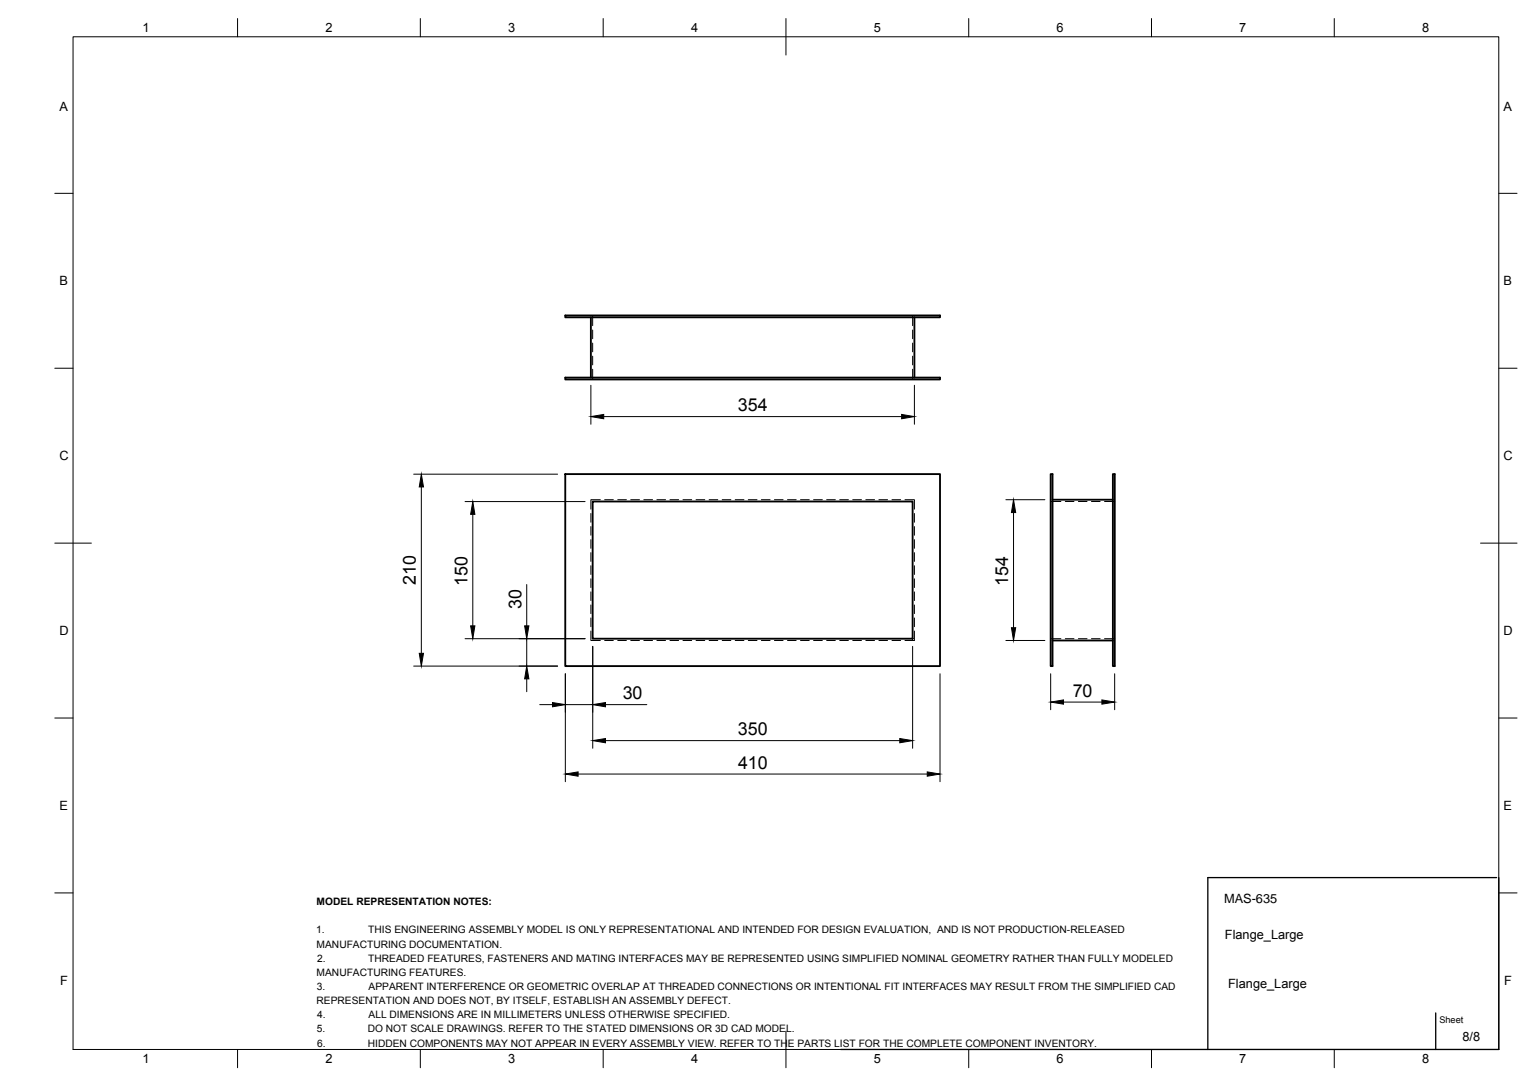
ISO-10303-21;
HEADER;
FILE_DESCRIPTION((''),'2;1');
FILE_NAME('Flange_Large.step','2026-10-09T12:34:24-07:00',(''),(''),'','','');
FILE_SCHEMA (('AUTOMOTIVE_DESIGN { 1 0 10303 214 3 1 1 }'));
ENDSEC;
DATA;
#10=MECHANICAL_DESIGN_GEOMETRIC_PRESENTATION_REPRESENTATION('',(#63),#3759);
#51=SHAPE_REPRESENTATION_RELATIONSHIP('SRR','None',#3792,#57) ;
#57=ADVANCED_BREP_SHAPE_REPRESENTATION('',(#69),#3757) ;
#63=STYLED_ITEM('',(#3827),#69) ;
#69=MANIFOLD_SOLID_BREP('Body1',#2267) ;
#133=FACE_BOUND('',#360,.T.) ;
#134=FACE_BOUND('',#362,.T.) ;
#135=FACE_BOUND('',#372,.T.) ;
#136=FACE_BOUND('',#374,.T.) ;
#221=FACE_OUTER_BOUND('',#355,.T.) ;
#222=FACE_OUTER_BOUND('',#356,.T.) ;
#223=FACE_OUTER_BOUND('',#357,.T.) ;
#224=FACE_OUTER_BOUND('',#358,.T.) ;
#225=FACE_OUTER_BOUND('',#359,.T.) ;
#226=FACE_OUTER_BOUND('',#361,.T.) ;
#227=FACE_OUTER_BOUND('',#363,.T.) ;
#228=FACE_OUTER_BOUND('',#364,.T.) ;
#229=FACE_OUTER_BOUND('',#365,.T.) ;
#230=FACE_OUTER_BOUND('',#366,.T.) ;
#231=FACE_OUTER_BOUND('',#367,.T.) ;
#232=FACE_OUTER_BOUND('',#368,.T.) ;
#233=FACE_OUTER_BOUND('',#369,.T.) ;
#234=FACE_OUTER_BOUND('',#370,.T.) ;
#235=FACE_OUTER_BOUND('',#371,.T.) ;
#236=FACE_OUTER_BOUND('',#373,.T.) ;
#237=FACE_OUTER_BOUND('',#375,.T.) ;
#238=FACE_OUTER_BOUND('',#376,.T.) ;
#239=FACE_OUTER_BOUND('',#377,.T.) ;
#240=FACE_OUTER_BOUND('',#378,.T.) ;
#355=EDGE_LOOP('',(#1847,#1848,#1849,#1850)) ;
#356=EDGE_LOOP('',(#1851,#1852,#1853,#1854)) ;
#357=EDGE_LOOP('',(#1855,#1856,#1857,#1858)) ;
#358=EDGE_LOOP('',(#1859,#1860,#1861,#1862)) ;
#359=EDGE_LOOP('',(#1863,#1864,#1865,#1866)) ;
#360=EDGE_LOOP('',(#1867,#1868,#1869,#1870)) ;
#361=EDGE_LOOP('',(#1871,#1872,#1873,#1874)) ;
#362=EDGE_LOOP('',(#1875,#1876,#1877,#1878)) ;
#363=EDGE_LOOP('',(#1879,#1880,#1881,#1882)) ;
#364=EDGE_LOOP('',(#1883,#1884,#1885,#1886)) ;
#365=EDGE_LOOP('',(#1887,#1888,#1889,#1890)) ;
#366=EDGE_LOOP('',(#1891,#1892,#1893,#1894)) ;
#367=EDGE_LOOP('',(#1895,#1896,#1897,#1898)) ;
#368=EDGE_LOOP('',(#1899,#1900,#1901,#1902)) ;
#369=EDGE_LOOP('',(#1903,#1904,#1905,#1906)) ;
#370=EDGE_LOOP('',(#1907,#1908,#1909,#1910)) ;
#371=EDGE_LOOP('',(#1911,#1912,#1913,#1914)) ;
#372=EDGE_LOOP('',(#1915,#1916,#1917,#1918)) ;
#373=EDGE_LOOP('',(#1919,#1920,#1921,#1922)) ;
#374=EDGE_LOOP('',(#1923,#1924,#1925,#1926)) ;
#375=EDGE_LOOP('',(#1927,#1928,#1929,#1930)) ;
#376=EDGE_LOOP('',(#1931,#1932,#1933,#1934)) ;
#377=EDGE_LOOP('',(#1935,#1936,#1937,#1938)) ;
#378=EDGE_LOOP('',(#1939,#1940,#1941,#1942)) ;
#575=LINE('',#3537,#843) ;
#576=LINE('',#3539,#844) ;
#577=LINE('',#3541,#845) ;
#578=LINE('',#3542,#846) ;
#579=LINE('',#3545,#847) ;
#580=LINE('',#3547,#848) ;
#581=LINE('',#3548,#849) ;
#582=LINE('',#3551,#850) ;
#583=LINE('',#3553,#851) ;
#584=LINE('',#3554,#852) ;
#585=LINE('',#3556,#853) ;
#586=LINE('',#3557,#854) ;
#587=LINE('',#3561,#855) ;
#588=LINE('',#3563,#856) ;
#589=LINE('',#3565,#857) ;
#590=LINE('',#3566,#858) ;
#591=LINE('',#3570,#859) ;
#592=LINE('',#3572,#860) ;
#593=LINE('',#3574,#861) ;
#594=LINE('',#3575,#862) ;
#595=LINE('',#3578,#863) ;
#596=LINE('',#3580,#864) ;
#597=LINE('',#3582,#865) ;
#598=LINE('',#3583,#866) ;
#599=LINE('',#3585,#867) ;
#600=LINE('',#3586,#868) ;
#601=LINE('',#3588,#869) ;
#602=LINE('',#3590,#870) ;
#603=LINE('',#3594,#871) ;
#604=LINE('',#3596,#872) ;
#605=LINE('',#3597,#873) ;
#606=LINE('',#3600,#874) ;
#607=LINE('',#3601,#875) ;
#608=LINE('',#3604,#876) ;
#609=LINE('',#3605,#877) ;
#610=LINE('',#3607,#878) ;
#611=LINE('',#3611,#879) ;
#612=LINE('',#3613,#880) ;
#613=LINE('',#3615,#881) ;
#614=LINE('',#3616,#882) ;
#615=LINE('',#3620,#883) ;
#616=LINE('',#3622,#884) ;
#617=LINE('',#3624,#885) ;
#618=LINE('',#3625,#886) ;
#619=LINE('',#3627,#887) ;
#620=LINE('',#3628,#888) ;
#621=LINE('',#3630,#889) ;
#622=LINE('',#3632,#890) ;
#843=VECTOR('',#2914,100.) ;
#844=VECTOR('',#2915,100.) ;
#845=VECTOR('',#2916,100.) ;
#846=VECTOR('',#2917,100.) ;
#847=VECTOR('',#2920,100.) ;
#848=VECTOR('',#2921,100.) ;
#849=VECTOR('',#2922,100.) ;
#850=VECTOR('',#2925,100.) ;
#851=VECTOR('',#2926,100.) ;
#852=VECTOR('',#2927,100.) ;
#853=VECTOR('',#2930,100.) ;
#854=VECTOR('',#2931,100.) ;
#855=VECTOR('',#2934,100.) ;
#856=VECTOR('',#2935,100.) ;
#857=VECTOR('',#2936,100.) ;
#858=VECTOR('',#2937,100.) ;
#859=VECTOR('',#2940,100.) ;
#860=VECTOR('',#2941,100.) ;
#861=VECTOR('',#2942,100.) ;
#862=VECTOR('',#2943,100.) ;
#863=VECTOR('',#2944,100.) ;
#864=VECTOR('',#2945,100.) ;
#865=VECTOR('',#2946,100.) ;
#866=VECTOR('',#2947,100.) ;
#867=VECTOR('',#2950,100.) ;
#868=VECTOR('',#2951,100.) ;
#869=VECTOR('',#2954,100.) ;
#870=VECTOR('',#2957,100.) ;
#871=VECTOR('',#2962,100.) ;
#872=VECTOR('',#2963,100.) ;
#873=VECTOR('',#2964,100.) ;
#874=VECTOR('',#2967,100.) ;
#875=VECTOR('',#2968,100.) ;
#876=VECTOR('',#2971,100.) ;
#877=VECTOR('',#2972,100.) ;
#878=VECTOR('',#2975,100.) ;
#879=VECTOR('',#2978,100.) ;
#880=VECTOR('',#2979,100.) ;
#881=VECTOR('',#2980,100.) ;
#882=VECTOR('',#2981,100.) ;
#883=VECTOR('',#2984,100.) ;
#884=VECTOR('',#2985,100.) ;
#885=VECTOR('',#2986,100.) ;
#886=VECTOR('',#2987,100.) ;
#887=VECTOR('',#2990,100.) ;
#888=VECTOR('',#2991,100.) ;
#889=VECTOR('',#2994,100.) ;
#890=VECTOR('',#2997,100.) ;
#1075=VERTEX_POINT('',#3535) ;
#1076=VERTEX_POINT('',#3536) ;
#1077=VERTEX_POINT('',#3538) ;
#1078=VERTEX_POINT('',#3540) ;
#1079=VERTEX_POINT('',#3544) ;
#1080=VERTEX_POINT('',#3546) ;
#1081=VERTEX_POINT('',#3550) ;
#1082=VERTEX_POINT('',#3552) ;
#1083=VERTEX_POINT('',#3559) ;
#1084=VERTEX_POINT('',#3560) ;
#1085=VERTEX_POINT('',#3562) ;
#1086=VERTEX_POINT('',#3564) ;
#1087=VERTEX_POINT('',#3568) ;
#1088=VERTEX_POINT('',#3569) ;
#1089=VERTEX_POINT('',#3571) ;
#1090=VERTEX_POINT('',#3573) ;
#1091=VERTEX_POINT('',#3576) ;
#1092=VERTEX_POINT('',#3577) ;
#1093=VERTEX_POINT('',#3579) ;
#1094=VERTEX_POINT('',#3581) ;
#1095=VERTEX_POINT('',#3593) ;
#1096=VERTEX_POINT('',#3595) ;
#1097=VERTEX_POINT('',#3599) ;
#1098=VERTEX_POINT('',#3603) ;
#1099=VERTEX_POINT('',#3609) ;
#1100=VERTEX_POINT('',#3610) ;
#1101=VERTEX_POINT('',#3612) ;
#1102=VERTEX_POINT('',#3614) ;
#1103=VERTEX_POINT('',#3618) ;
#1104=VERTEX_POINT('',#3619) ;
#1105=VERTEX_POINT('',#3621) ;
#1106=VERTEX_POINT('',#3623) ;
#1343=EDGE_CURVE('',#1075,#1076,#575,.T.) ;
#1344=EDGE_CURVE('',#1075,#1077,#576,.T.) ;
#1345=EDGE_CURVE('',#1078,#1077,#577,.T.) ;
#1346=EDGE_CURVE('',#1076,#1078,#578,.T.) ;
#1347=EDGE_CURVE('',#1076,#1079,#579,.T.) ;
#1348=EDGE_CURVE('',#1080,#1078,#580,.T.) ;
#1349=EDGE_CURVE('',#1079,#1080,#581,.T.) ;
#1350=EDGE_CURVE('',#1079,#1081,#582,.T.) ;
#1351=EDGE_CURVE('',#1082,#1080,#583,.T.) ;
#1352=EDGE_CURVE('',#1081,#1082,#584,.T.) ;
#1353=EDGE_CURVE('',#1081,#1075,#585,.T.) ;
#1354=EDGE_CURVE('',#1077,#1082,#586,.T.) ;
#1355=EDGE_CURVE('',#1083,#1084,#587,.T.) ;
#1356=EDGE_CURVE('',#1084,#1085,#588,.T.) ;
#1357=EDGE_CURVE('',#1085,#1086,#589,.T.) ;
#1358=EDGE_CURVE('',#1086,#1083,#590,.T.) ;
#1359=EDGE_CURVE('',#1087,#1088,#591,.T.) ;
#1360=EDGE_CURVE('',#1089,#1087,#592,.T.) ;
#1361=EDGE_CURVE('',#1090,#1089,#593,.T.) ;
#1362=EDGE_CURVE('',#1088,#1090,#594,.T.) ;
#1363=EDGE_CURVE('',#1091,#1092,#595,.T.) ;
#1364=EDGE_CURVE('',#1092,#1093,#596,.T.) ;
#1365=EDGE_CURVE('',#1093,#1094,#597,.T.) ;
#1366=EDGE_CURVE('',#1094,#1091,#598,.T.) ;
#1367=EDGE_CURVE('',#1084,#1088,#599,.T.) ;
#1368=EDGE_CURVE('',#1083,#1087,#600,.T.) ;
#1369=EDGE_CURVE('',#1085,#1090,#601,.T.) ;
#1370=EDGE_CURVE('',#1086,#1089,#602,.T.) ;
#1371=EDGE_CURVE('',#1095,#1092,#603,.T.) ;
#1372=EDGE_CURVE('',#1096,#1091,#604,.T.) ;
#1373=EDGE_CURVE('',#1096,#1095,#605,.T.) ;
#1374=EDGE_CURVE('',#1097,#1093,#606,.T.) ;
#1375=EDGE_CURVE('',#1095,#1097,#607,.T.) ;
#1376=EDGE_CURVE('',#1098,#1094,#608,.T.) ;
#1377=EDGE_CURVE('',#1097,#1098,#609,.T.) ;
#1378=EDGE_CURVE('',#1098,#1096,#610,.T.) ;
#1379=EDGE_CURVE('',#1099,#1100,#611,.T.) ;
#1380=EDGE_CURVE('',#1100,#1101,#612,.T.) ;
#1381=EDGE_CURVE('',#1101,#1102,#613,.T.) ;
#1382=EDGE_CURVE('',#1102,#1099,#614,.T.) ;
#1383=EDGE_CURVE('',#1103,#1104,#615,.T.) ;
#1384=EDGE_CURVE('',#1105,#1103,#616,.T.) ;
#1385=EDGE_CURVE('',#1106,#1105,#617,.T.) ;
#1386=EDGE_CURVE('',#1104,#1106,#618,.T.) ;
#1387=EDGE_CURVE('',#1103,#1099,#619,.T.) ;
#1388=EDGE_CURVE('',#1104,#1100,#620,.T.) ;
#1389=EDGE_CURVE('',#1105,#1102,#621,.T.) ;
#1390=EDGE_CURVE('',#1106,#1101,#622,.T.) ;
#1847=ORIENTED_EDGE('',*,*,#1343,.F.) ;
#1848=ORIENTED_EDGE('',*,*,#1344,.T.) ;
#1849=ORIENTED_EDGE('',*,*,#1345,.F.) ;
#1850=ORIENTED_EDGE('',*,*,#1346,.F.) ;
#1851=ORIENTED_EDGE('',*,*,#1347,.F.) ;
#1852=ORIENTED_EDGE('',*,*,#1346,.T.) ;
#1853=ORIENTED_EDGE('',*,*,#1348,.F.) ;
#1854=ORIENTED_EDGE('',*,*,#1349,.F.) ;
#1855=ORIENTED_EDGE('',*,*,#1350,.F.) ;
#1856=ORIENTED_EDGE('',*,*,#1349,.T.) ;
#1857=ORIENTED_EDGE('',*,*,#1351,.F.) ;
#1858=ORIENTED_EDGE('',*,*,#1352,.F.) ;
#1859=ORIENTED_EDGE('',*,*,#1353,.F.) ;
#1860=ORIENTED_EDGE('',*,*,#1352,.T.) ;
#1861=ORIENTED_EDGE('',*,*,#1354,.F.) ;
#1862=ORIENTED_EDGE('',*,*,#1344,.F.) ;
#1863=ORIENTED_EDGE('',*,*,#1355,.T.) ;
#1864=ORIENTED_EDGE('',*,*,#1356,.T.) ;
#1865=ORIENTED_EDGE('',*,*,#1357,.T.) ;
#1866=ORIENTED_EDGE('',*,*,#1358,.T.) ;
#1867=ORIENTED_EDGE('',*,*,#1348,.T.) ;
#1868=ORIENTED_EDGE('',*,*,#1345,.T.) ;
#1869=ORIENTED_EDGE('',*,*,#1354,.T.) ;
#1870=ORIENTED_EDGE('',*,*,#1351,.T.) ;
#1871=ORIENTED_EDGE('',*,*,#1359,.F.) ;
#1872=ORIENTED_EDGE('',*,*,#1360,.F.) ;
#1873=ORIENTED_EDGE('',*,*,#1361,.F.) ;
#1874=ORIENTED_EDGE('',*,*,#1362,.F.) ;
#1875=ORIENTED_EDGE('',*,*,#1363,.T.) ;
#1876=ORIENTED_EDGE('',*,*,#1364,.T.) ;
#1877=ORIENTED_EDGE('',*,*,#1365,.T.) ;
#1878=ORIENTED_EDGE('',*,*,#1366,.T.) ;
#1879=ORIENTED_EDGE('',*,*,#1359,.T.) ;
#1880=ORIENTED_EDGE('',*,*,#1367,.F.) ;
#1881=ORIENTED_EDGE('',*,*,#1355,.F.) ;
#1882=ORIENTED_EDGE('',*,*,#1368,.T.) ;
#1883=ORIENTED_EDGE('',*,*,#1362,.T.) ;
#1884=ORIENTED_EDGE('',*,*,#1369,.F.) ;
#1885=ORIENTED_EDGE('',*,*,#1356,.F.) ;
#1886=ORIENTED_EDGE('',*,*,#1367,.T.) ;
#1887=ORIENTED_EDGE('',*,*,#1361,.T.) ;
#1888=ORIENTED_EDGE('',*,*,#1370,.F.) ;
#1889=ORIENTED_EDGE('',*,*,#1357,.F.) ;
#1890=ORIENTED_EDGE('',*,*,#1369,.T.) ;
#1891=ORIENTED_EDGE('',*,*,#1360,.T.) ;
#1892=ORIENTED_EDGE('',*,*,#1368,.F.) ;
#1893=ORIENTED_EDGE('',*,*,#1358,.F.) ;
#1894=ORIENTED_EDGE('',*,*,#1370,.T.) ;
#1895=ORIENTED_EDGE('',*,*,#1371,.T.) ;
#1896=ORIENTED_EDGE('',*,*,#1363,.F.) ;
#1897=ORIENTED_EDGE('',*,*,#1372,.F.) ;
#1898=ORIENTED_EDGE('',*,*,#1373,.T.) ;
#1899=ORIENTED_EDGE('',*,*,#1374,.T.) ;
#1900=ORIENTED_EDGE('',*,*,#1364,.F.) ;
#1901=ORIENTED_EDGE('',*,*,#1371,.F.) ;
#1902=ORIENTED_EDGE('',*,*,#1375,.T.) ;
#1903=ORIENTED_EDGE('',*,*,#1376,.T.) ;
#1904=ORIENTED_EDGE('',*,*,#1365,.F.) ;
#1905=ORIENTED_EDGE('',*,*,#1374,.F.) ;
#1906=ORIENTED_EDGE('',*,*,#1377,.T.) ;
#1907=ORIENTED_EDGE('',*,*,#1372,.T.) ;
#1908=ORIENTED_EDGE('',*,*,#1366,.F.) ;
#1909=ORIENTED_EDGE('',*,*,#1376,.F.) ;
#1910=ORIENTED_EDGE('',*,*,#1378,.T.) ;
#1911=ORIENTED_EDGE('',*,*,#1379,.T.) ;
#1912=ORIENTED_EDGE('',*,*,#1380,.T.) ;
#1913=ORIENTED_EDGE('',*,*,#1381,.T.) ;
#1914=ORIENTED_EDGE('',*,*,#1382,.T.) ;
#1915=ORIENTED_EDGE('',*,*,#1375,.F.) ;
#1916=ORIENTED_EDGE('',*,*,#1373,.F.) ;
#1917=ORIENTED_EDGE('',*,*,#1378,.F.) ;
#1918=ORIENTED_EDGE('',*,*,#1377,.F.) ;
#1919=ORIENTED_EDGE('',*,*,#1383,.F.) ;
#1920=ORIENTED_EDGE('',*,*,#1384,.F.) ;
#1921=ORIENTED_EDGE('',*,*,#1385,.F.) ;
#1922=ORIENTED_EDGE('',*,*,#1386,.F.) ;
#1923=ORIENTED_EDGE('',*,*,#1353,.T.) ;
#1924=ORIENTED_EDGE('',*,*,#1343,.T.) ;
#1925=ORIENTED_EDGE('',*,*,#1347,.T.) ;
#1926=ORIENTED_EDGE('',*,*,#1350,.T.) ;
#1927=ORIENTED_EDGE('',*,*,#1379,.F.) ;
#1928=ORIENTED_EDGE('',*,*,#1387,.F.) ;
#1929=ORIENTED_EDGE('',*,*,#1383,.T.) ;
#1930=ORIENTED_EDGE('',*,*,#1388,.T.) ;
#1931=ORIENTED_EDGE('',*,*,#1382,.F.) ;
#1932=ORIENTED_EDGE('',*,*,#1389,.F.) ;
#1933=ORIENTED_EDGE('',*,*,#1384,.T.) ;
#1934=ORIENTED_EDGE('',*,*,#1387,.T.) ;
#1935=ORIENTED_EDGE('',*,*,#1381,.F.) ;
#1936=ORIENTED_EDGE('',*,*,#1390,.F.) ;
#1937=ORIENTED_EDGE('',*,*,#1385,.T.) ;
#1938=ORIENTED_EDGE('',*,*,#1389,.T.) ;
#1939=ORIENTED_EDGE('',*,*,#1380,.F.) ;
#1940=ORIENTED_EDGE('',*,*,#1388,.F.) ;
#1941=ORIENTED_EDGE('',*,*,#1386,.T.) ;
#1942=ORIENTED_EDGE('',*,*,#1390,.T.) ;
#2103=PLANE('',#2454) ;
#2104=PLANE('',#2455) ;
#2105=PLANE('',#2456) ;
#2106=PLANE('',#2457) ;
#2107=PLANE('',#2458) ;
#2108=PLANE('',#2459) ;
#2109=PLANE('',#2460) ;
#2110=PLANE('',#2461) ;
#2111=PLANE('',#2462) ;
#2112=PLANE('',#2463) ;
#2113=PLANE('',#2464) ;
#2114=PLANE('',#2465) ;
#2115=PLANE('',#2466) ;
#2116=PLANE('',#2467) ;
#2117=PLANE('',#2468) ;
#2118=PLANE('',#2469) ;
#2119=PLANE('',#2470) ;
#2120=PLANE('',#2471) ;
#2121=PLANE('',#2472) ;
#2122=PLANE('',#2473) ;
#2223=ADVANCED_FACE('',(#221),#2103,.F.) ;
#2224=ADVANCED_FACE('',(#222),#2104,.F.) ;
#2225=ADVANCED_FACE('',(#223),#2105,.F.) ;
#2226=ADVANCED_FACE('',(#224),#2106,.F.) ;
#2227=ADVANCED_FACE('',(#225,#133),#2107,.T.) ;
#2228=ADVANCED_FACE('',(#226,#134),#2108,.F.) ;
#2229=ADVANCED_FACE('',(#227),#2109,.F.) ;
#2230=ADVANCED_FACE('',(#228),#2110,.F.) ;
#2231=ADVANCED_FACE('',(#229),#2111,.F.) ;
#2232=ADVANCED_FACE('',(#230),#2112,.F.) ;
#2233=ADVANCED_FACE('',(#231),#2113,.T.) ;
#2234=ADVANCED_FACE('',(#232),#2114,.T.) ;
#2235=ADVANCED_FACE('',(#233),#2115,.T.) ;
#2236=ADVANCED_FACE('',(#234),#2116,.T.) ;
#2237=ADVANCED_FACE('',(#235,#135),#2117,.T.) ;
#2238=ADVANCED_FACE('',(#236,#136),#2118,.F.) ;
#2239=ADVANCED_FACE('',(#237),#2119,.T.) ;
#2240=ADVANCED_FACE('',(#238),#2120,.T.) ;
#2241=ADVANCED_FACE('',(#239),#2121,.T.) ;
#2242=ADVANCED_FACE('',(#240),#2122,.T.) ;
#2267=CLOSED_SHELL('',(#2223,#2224,#2225,#2226,#2227,#2228,#2229,#2230,
#2231,#2232,#2233,#2234,#2235,#2236,#2237,#2238,#2239,#2240,#2241,#2242)) ;
#2453=AXIS2_PLACEMENT_3D('',#3533,#2910,#2911) ;
#2454=AXIS2_PLACEMENT_3D('',#3534,#2912,#2913) ;
#2455=AXIS2_PLACEMENT_3D('',#3543,#2918,#2919) ;
#2456=AXIS2_PLACEMENT_3D('',#3549,#2923,#2924) ;
#2457=AXIS2_PLACEMENT_3D('',#3555,#2928,#2929) ;
#2458=AXIS2_PLACEMENT_3D('',#3558,#2932,#2933) ;
#2459=AXIS2_PLACEMENT_3D('',#3567,#2938,#2939) ;
#2460=AXIS2_PLACEMENT_3D('',#3584,#2948,#2949) ;
#2461=AXIS2_PLACEMENT_3D('',#3587,#2952,#2953) ;
#2462=AXIS2_PLACEMENT_3D('',#3589,#2955,#2956) ;
#2463=AXIS2_PLACEMENT_3D('',#3591,#2958,#2959) ;
#2464=AXIS2_PLACEMENT_3D('',#3592,#2960,#2961) ;
#2465=AXIS2_PLACEMENT_3D('',#3598,#2965,#2966) ;
#2466=AXIS2_PLACEMENT_3D('',#3602,#2969,#2970) ;
#2467=AXIS2_PLACEMENT_3D('',#3606,#2973,#2974) ;
#2468=AXIS2_PLACEMENT_3D('',#3608,#2976,#2977) ;
#2469=AXIS2_PLACEMENT_3D('',#3617,#2982,#2983) ;
#2470=AXIS2_PLACEMENT_3D('',#3626,#2988,#2989) ;
#2471=AXIS2_PLACEMENT_3D('',#3629,#2992,#2993) ;
#2472=AXIS2_PLACEMENT_3D('',#3631,#2995,#2996) ;
#2473=AXIS2_PLACEMENT_3D('',#3633,#2998,#2999) ;
#2910=DIRECTION('axis',(0.,0.,1.)) ;
#2911=DIRECTION('refdir',(1.,0.,0.)) ;
#2912=DIRECTION('center_axis',(-1.,-3.70074341541719E-16,0.)) ;
#2913=DIRECTION('ref_axis',(3.70074341541719E-16,-1.,0.)) ;
#2914=DIRECTION('',(-3.70074341541719E-16,1.,0.)) ;
#2915=DIRECTION('',(0.,0.,-1.)) ;
#2916=DIRECTION('',(3.70074341541719E-16,-1.,0.)) ;
#2917=DIRECTION('',(0.,0.,-1.)) ;
#2918=DIRECTION('center_axis',(0.,-1.,0.)) ;
#2919=DIRECTION('ref_axis',(0.,0.,-1.)) ;
#2920=DIRECTION('',(-1.,0.,0.)) ;
#2921=DIRECTION('',(1.,0.,0.)) ;
#2922=DIRECTION('',(0.,0.,-1.)) ;
#2923=DIRECTION('center_axis',(1.,3.70074341541719E-16,0.)) ;
#2924=DIRECTION('ref_axis',(-3.70074341541719E-16,1.,0.)) ;
#2925=DIRECTION('',(3.70074341541719E-16,-1.,0.)) ;
#2926=DIRECTION('',(-3.70074341541719E-16,1.,0.)) ;
#2927=DIRECTION('',(0.,0.,-1.)) ;
#2928=DIRECTION('center_axis',(0.,1.,0.)) ;
#2929=DIRECTION('ref_axis',(0.,0.,1.)) ;
#2930=DIRECTION('',(1.,0.,0.)) ;
#2931=DIRECTION('',(-1.,0.,0.)) ;
#2932=DIRECTION('center_axis',(0.,0.,1.)) ;
#2933=DIRECTION('ref_axis',(1.,0.,0.)) ;
#2934=DIRECTION('',(-3.70074341541719E-16,1.,0.)) ;
#2935=DIRECTION('',(-1.,0.,0.)) ;
#2936=DIRECTION('',(3.70074341541719E-16,-1.,0.)) ;
#2937=DIRECTION('',(1.,0.,0.)) ;
#2938=DIRECTION('center_axis',(0.,0.,1.)) ;
#2939=DIRECTION('ref_axis',(1.,0.,0.)) ;
#2940=DIRECTION('',(-3.70074341541719E-16,1.,0.)) ;
#2941=DIRECTION('',(1.,0.,0.)) ;
#2942=DIRECTION('',(3.70074341541719E-16,-1.,0.)) ;
#2943=DIRECTION('',(-1.,0.,0.)) ;
#2944=DIRECTION('',(-3.70074341541719E-16,1.,0.)) ;
#2945=DIRECTION('',(-1.,0.,0.)) ;
#2946=DIRECTION('',(3.70074341541719E-16,-1.,0.)) ;
#2947=DIRECTION('',(1.,0.,0.)) ;
#2948=DIRECTION('center_axis',(-1.,-3.70074341541719E-16,0.)) ;
#2949=DIRECTION('ref_axis',(3.70074341541719E-16,-1.,0.)) ;
#2950=DIRECTION('',(0.,0.,-1.)) ;
#2951=DIRECTION('',(0.,0.,-1.)) ;
#2952=DIRECTION('center_axis',(0.,-1.,0.)) ;
#2953=DIRECTION('ref_axis',(0.,0.,-1.)) ;
#2954=DIRECTION('',(0.,0.,-1.)) ;
#2955=DIRECTION('center_axis',(1.,3.70074341541719E-16,0.)) ;
#2956=DIRECTION('ref_axis',(-3.70074341541719E-16,1.,0.)) ;
#2957=DIRECTION('',(0.,0.,-1.)) ;
#2958=DIRECTION('center_axis',(0.,1.,0.)) ;
#2959=DIRECTION('ref_axis',(0.,0.,1.)) ;
#2960=DIRECTION('center_axis',(-1.,-3.70074341541719E-16,0.)) ;
#2961=DIRECTION('ref_axis',(3.70074341541719E-16,-1.,0.)) ;
#2962=DIRECTION('',(0.,0.,-1.)) ;
#2963=DIRECTION('',(0.,0.,-1.)) ;
#2964=DIRECTION('',(-3.70074341541719E-16,1.,0.)) ;
#2965=DIRECTION('center_axis',(0.,-1.,0.)) ;
#2966=DIRECTION('ref_axis',(0.,0.,-1.)) ;
#2967=DIRECTION('',(0.,0.,-1.)) ;
#2968=DIRECTION('',(-1.,0.,0.)) ;
#2969=DIRECTION('center_axis',(1.,3.70074341541719E-16,0.)) ;
#2970=DIRECTION('ref_axis',(-3.70074341541719E-16,1.,0.)) ;
#2971=DIRECTION('',(0.,0.,-1.)) ;
#2972=DIRECTION('',(3.70074341541719E-16,-1.,0.)) ;
#2973=DIRECTION('center_axis',(0.,1.,0.)) ;
#2974=DIRECTION('ref_axis',(0.,0.,1.)) ;
#2975=DIRECTION('',(1.,0.,0.)) ;
#2976=DIRECTION('center_axis',(0.,0.,1.)) ;
#2977=DIRECTION('ref_axis',(1.,0.,0.)) ;
#2978=DIRECTION('',(3.70074341541719E-16,-1.,0.)) ;
#2979=DIRECTION('',(1.,0.,0.)) ;
#2980=DIRECTION('',(-3.70074341541719E-16,1.,0.)) ;
#2981=DIRECTION('',(-1.,0.,0.)) ;
#2982=DIRECTION('center_axis',(0.,0.,1.)) ;
#2983=DIRECTION('ref_axis',(1.,0.,0.)) ;
#2984=DIRECTION('',(3.70074341541719E-16,-1.,0.)) ;
#2985=DIRECTION('',(-1.,0.,0.)) ;
#2986=DIRECTION('',(-3.70074341541719E-16,1.,0.)) ;
#2987=DIRECTION('',(1.,0.,0.)) ;
#2988=DIRECTION('center_axis',(-1.,-3.70074341541719E-16,0.)) ;
#2989=DIRECTION('ref_axis',(3.70074341541719E-16,-1.,0.)) ;
#2990=DIRECTION('',(0.,0.,1.)) ;
#2991=DIRECTION('',(0.,0.,1.)) ;
#2992=DIRECTION('center_axis',(0.,1.,0.)) ;
#2993=DIRECTION('ref_axis',(0.,0.,1.)) ;
#2994=DIRECTION('',(0.,0.,1.)) ;
#2995=DIRECTION('center_axis',(1.,3.70074341541719E-16,0.)) ;
#2996=DIRECTION('ref_axis',(-3.70074341541719E-16,1.,0.)) ;
#2997=DIRECTION('',(0.,0.,1.)) ;
#2998=DIRECTION('center_axis',(0.,-1.,0.)) ;
#2999=DIRECTION('ref_axis',(0.,0.,-1.)) ;
#3533=CARTESIAN_POINT('',(0.,0.,0.)) ;
#3534=CARTESIAN_POINT('Origin',(17.7,7.5,7.)) ;
#3535=CARTESIAN_POINT('',(17.7,-7.7,6.8)) ;
#3536=CARTESIAN_POINT('',(17.7,7.7,6.8)) ;
#3537=CARTESIAN_POINT('',(17.7,7.5,6.8)) ;
#3538=CARTESIAN_POINT('',(17.7,-7.7,0.2)) ;
#3539=CARTESIAN_POINT('',(17.7,-7.7,7.)) ;
#3540=CARTESIAN_POINT('',(17.7,7.7,0.2)) ;
#3541=CARTESIAN_POINT('',(17.7,6.55031584528842E-15,0.2)) ;
#3542=CARTESIAN_POINT('',(17.7,7.7,7.)) ;
#3543=CARTESIAN_POINT('Origin',(-17.5,7.7,7.)) ;
#3544=CARTESIAN_POINT('',(-17.7,7.7,6.8)) ;
#3545=CARTESIAN_POINT('',(-17.5,7.7,6.8)) ;
#3546=CARTESIAN_POINT('',(-17.7,7.7,0.2)) ;
#3547=CARTESIAN_POINT('',(0.,7.7,0.2)) ;
#3548=CARTESIAN_POINT('',(-17.7,7.7,7.)) ;
#3549=CARTESIAN_POINT('Origin',(-17.7,7.5,7.)) ;
#3550=CARTESIAN_POINT('',(-17.7,-7.7,6.8)) ;
#3551=CARTESIAN_POINT('',(-17.7,7.5,6.8)) ;
#3552=CARTESIAN_POINT('',(-17.7,-7.7,0.2)) ;
#3553=CARTESIAN_POINT('',(-17.7,-6.55031584528843E-15,0.2)) ;
#3554=CARTESIAN_POINT('',(-17.7,-7.7,7.)) ;
#3555=CARTESIAN_POINT('Origin',(-17.5,-7.7,7.)) ;
#3556=CARTESIAN_POINT('',(-17.5,-7.7,6.8)) ;
#3557=CARTESIAN_POINT('',(0.,-7.7,0.2)) ;
#3558=CARTESIAN_POINT('Origin',(0.,0.,0.2)) ;
#3559=CARTESIAN_POINT('',(20.5,-10.5,0.2)) ;
#3560=CARTESIAN_POINT('',(20.5,10.5,0.2)) ;
#3561=CARTESIAN_POINT('',(20.5,7.5,0.2)) ;
#3562=CARTESIAN_POINT('',(-20.5,10.5,0.2)) ;
#3563=CARTESIAN_POINT('',(-17.5,10.5,0.2)) ;
#3564=CARTESIAN_POINT('',(-20.5,-10.5,0.2)) ;
#3565=CARTESIAN_POINT('',(-20.5,7.5,0.2)) ;
#3566=CARTESIAN_POINT('',(-17.5,-10.5,0.2)) ;
#3567=CARTESIAN_POINT('Origin',(0.,0.,0.)) ;
#3568=CARTESIAN_POINT('',(20.5,-10.5,0.)) ;
#3569=CARTESIAN_POINT('',(20.5,10.5,0.)) ;
#3570=CARTESIAN_POINT('',(20.5,7.5,0.)) ;
#3571=CARTESIAN_POINT('',(-20.5,-10.5,0.)) ;
#3572=CARTESIAN_POINT('',(-17.5,-10.5,0.)) ;
#3573=CARTESIAN_POINT('',(-20.5,10.5,0.)) ;
#3574=CARTESIAN_POINT('',(-20.5,7.5,0.)) ;
#3575=CARTESIAN_POINT('',(-17.5,10.5,0.)) ;
#3576=CARTESIAN_POINT('',(17.5,-7.5,0.)) ;
#3577=CARTESIAN_POINT('',(17.5,7.5,0.)) ;
#3578=CARTESIAN_POINT('',(17.5,7.5,0.)) ;
#3579=CARTESIAN_POINT('',(-17.5,7.5,0.)) ;
#3580=CARTESIAN_POINT('',(-17.5,7.5,0.)) ;
#3581=CARTESIAN_POINT('',(-17.5,-7.5,0.)) ;
#3582=CARTESIAN_POINT('',(-17.5,7.5,0.)) ;
#3583=CARTESIAN_POINT('',(-17.5,-7.5,0.)) ;
#3584=CARTESIAN_POINT('Origin',(20.5,7.5,0.2)) ;
#3585=CARTESIAN_POINT('',(20.5,10.5,0.2)) ;
#3586=CARTESIAN_POINT('',(20.5,-10.5,0.2)) ;
#3587=CARTESIAN_POINT('Origin',(-17.5,10.5,0.2)) ;
#3588=CARTESIAN_POINT('',(-20.5,10.5,0.2)) ;
#3589=CARTESIAN_POINT('Origin',(-20.5,7.5,0.2)) ;
#3590=CARTESIAN_POINT('',(-20.5,-10.5,0.2)) ;
#3591=CARTESIAN_POINT('Origin',(-17.5,-10.5,0.2)) ;
#3592=CARTESIAN_POINT('Origin',(17.5,7.5,0.2)) ;
#3593=CARTESIAN_POINT('',(17.5,7.5,7.)) ;
#3594=CARTESIAN_POINT('',(17.5,7.5,0.2)) ;
#3595=CARTESIAN_POINT('',(17.5,-7.5,7.)) ;
#3596=CARTESIAN_POINT('',(17.5,-7.5,0.2)) ;
#3597=CARTESIAN_POINT('',(17.5,7.5,7.)) ;
#3598=CARTESIAN_POINT('Origin',(-17.5,7.5,0.2)) ;
#3599=CARTESIAN_POINT('',(-17.5,7.5,7.)) ;
#3600=CARTESIAN_POINT('',(-17.5,7.5,0.2)) ;
#3601=CARTESIAN_POINT('',(-17.5,7.5,7.)) ;
#3602=CARTESIAN_POINT('Origin',(-17.5,7.5,0.2)) ;
#3603=CARTESIAN_POINT('',(-17.5,-7.5,7.)) ;
#3604=CARTESIAN_POINT('',(-17.5,-7.5,0.2)) ;
#3605=CARTESIAN_POINT('',(-17.5,7.5,7.)) ;
#3606=CARTESIAN_POINT('Origin',(-17.5,-7.5,0.2)) ;
#3607=CARTESIAN_POINT('',(-17.5,-7.5,7.)) ;
#3608=CARTESIAN_POINT('Origin',(0.,0.,7.)) ;
#3609=CARTESIAN_POINT('',(-20.5,10.5,7.)) ;
#3610=CARTESIAN_POINT('',(-20.5,-10.5,7.)) ;
#3611=CARTESIAN_POINT('',(-20.5,7.5,7.)) ;
#3612=CARTESIAN_POINT('',(20.5,-10.5,7.)) ;
#3613=CARTESIAN_POINT('',(-17.5,-10.5,7.)) ;
#3614=CARTESIAN_POINT('',(20.5,10.5,7.)) ;
#3615=CARTESIAN_POINT('',(20.5,-7.5,7.)) ;
#3616=CARTESIAN_POINT('',(17.5,10.5,7.)) ;
#3617=CARTESIAN_POINT('Origin',(0.,0.,6.8)) ;
#3618=CARTESIAN_POINT('',(-20.5,10.5,6.8)) ;
#3619=CARTESIAN_POINT('',(-20.5,-10.5,6.8)) ;
#3620=CARTESIAN_POINT('',(-20.5,7.5,6.8)) ;
#3621=CARTESIAN_POINT('',(20.5,10.5,6.8)) ;
#3622=CARTESIAN_POINT('',(17.5,10.5,6.8)) ;
#3623=CARTESIAN_POINT('',(20.5,-10.5,6.8)) ;
#3624=CARTESIAN_POINT('',(20.5,-7.5,6.8)) ;
#3625=CARTESIAN_POINT('',(-17.5,-10.5,6.8)) ;
#3626=CARTESIAN_POINT('Origin',(-20.5,7.5,6.8)) ;
#3627=CARTESIAN_POINT('',(-20.5,10.5,6.8)) ;
#3628=CARTESIAN_POINT('',(-20.5,-10.5,6.8)) ;
#3629=CARTESIAN_POINT('Origin',(17.5,10.5,6.8)) ;
#3630=CARTESIAN_POINT('',(20.5,10.5,6.8)) ;
#3631=CARTESIAN_POINT('Origin',(20.5,-7.5,6.8)) ;
#3632=CARTESIAN_POINT('',(20.5,-10.5,6.8)) ;
#3633=CARTESIAN_POINT('Origin',(-17.5,-10.5,6.8)) ;
#3749=UNCERTAINTY_MEASURE_WITH_UNIT(LENGTH_MEASURE(0.001),#3760,
'DISTANCE_ACCURACY_VALUE',
'Maximum model space distance between geometric entities at asserted c
onnectivities') ;
#3751=UNCERTAINTY_MEASURE_WITH_UNIT(LENGTH_MEASURE(0.001),#3760,
'DISTANCE_ACCURACY_VALUE',
'Maximum model space distance between geometric entities at asserted c
onnectivities') ;
#3757=(
GEOMETRIC_REPRESENTATION_CONTEXT(3)
GLOBAL_UNCERTAINTY_ASSIGNED_CONTEXT((#3749))
GLOBAL_UNIT_ASSIGNED_CONTEXT((#3760,#3762,#3763))
REPRESENTATION_CONTEXT('','3D')
) ;
#3759=(
GEOMETRIC_REPRESENTATION_CONTEXT(3)
GLOBAL_UNCERTAINTY_ASSIGNED_CONTEXT((#3751))
GLOBAL_UNIT_ASSIGNED_CONTEXT((#3760,#3762,#3763))
REPRESENTATION_CONTEXT('','3D')
) ;
#3760=(
LENGTH_UNIT()
NAMED_UNIT(*)
SI_UNIT(.CENTI.,.METRE.)
) ;
#3762=(
NAMED_UNIT(*)
PLANE_ANGLE_UNIT()
SI_UNIT($,.RADIAN.)
) ;
#3763=(
NAMED_UNIT(*)
SI_UNIT($,.STERADIAN.)
SOLID_ANGLE_UNIT()
) ;
#3769=SHAPE_DEFINITION_REPRESENTATION(#3776,#3792) ;
#3776=PRODUCT_DEFINITION_SHAPE('',$,#3800) ;
#3792=SHAPE_REPRESENTATION('',(#2453),#3757) ;
#3794=PRODUCT_DEFINITION_CONTEXT('part definition',#3817,'design') ;
#3800=PRODUCT_DEFINITION('Flange_Large','Flange_Large',#3807,
#3794) ;
#3807=PRODUCT_DEFINITION_FORMATION('',$,#3824) ;
#3817=APPLICATION_CONTEXT(
'Core Data for Automotive Mechanical Design Process') ;
#3818=PRODUCT_CONTEXT('part definition',#3817,'mechanical') ;
#3824=PRODUCT('Flange_Large','Flange_Large',$,(#3818)) ;
#3827=PRESENTATION_STYLE_ASSIGNMENT((#3829)) ;
#3829=SURFACE_STYLE_USAGE(.BOTH.,#3831) ;
#3831=SURFACE_SIDE_STYLE('',(#3833)) ;
#3833=SURFACE_STYLE_FILL_AREA(#3835) ;
#3835=FILL_AREA_STYLE('Opaque(179,179,179)',(#3837)) ;
#3837=FILL_AREA_STYLE_COLOUR('Opaque(179,179,179)',#3839) ;
#3839=COLOUR_RGB('Opaque(179,179,179)', 0.09019608, 0.27058824, 0.51372549) ;
ENDSEC;
END-ISO-10303-21;
